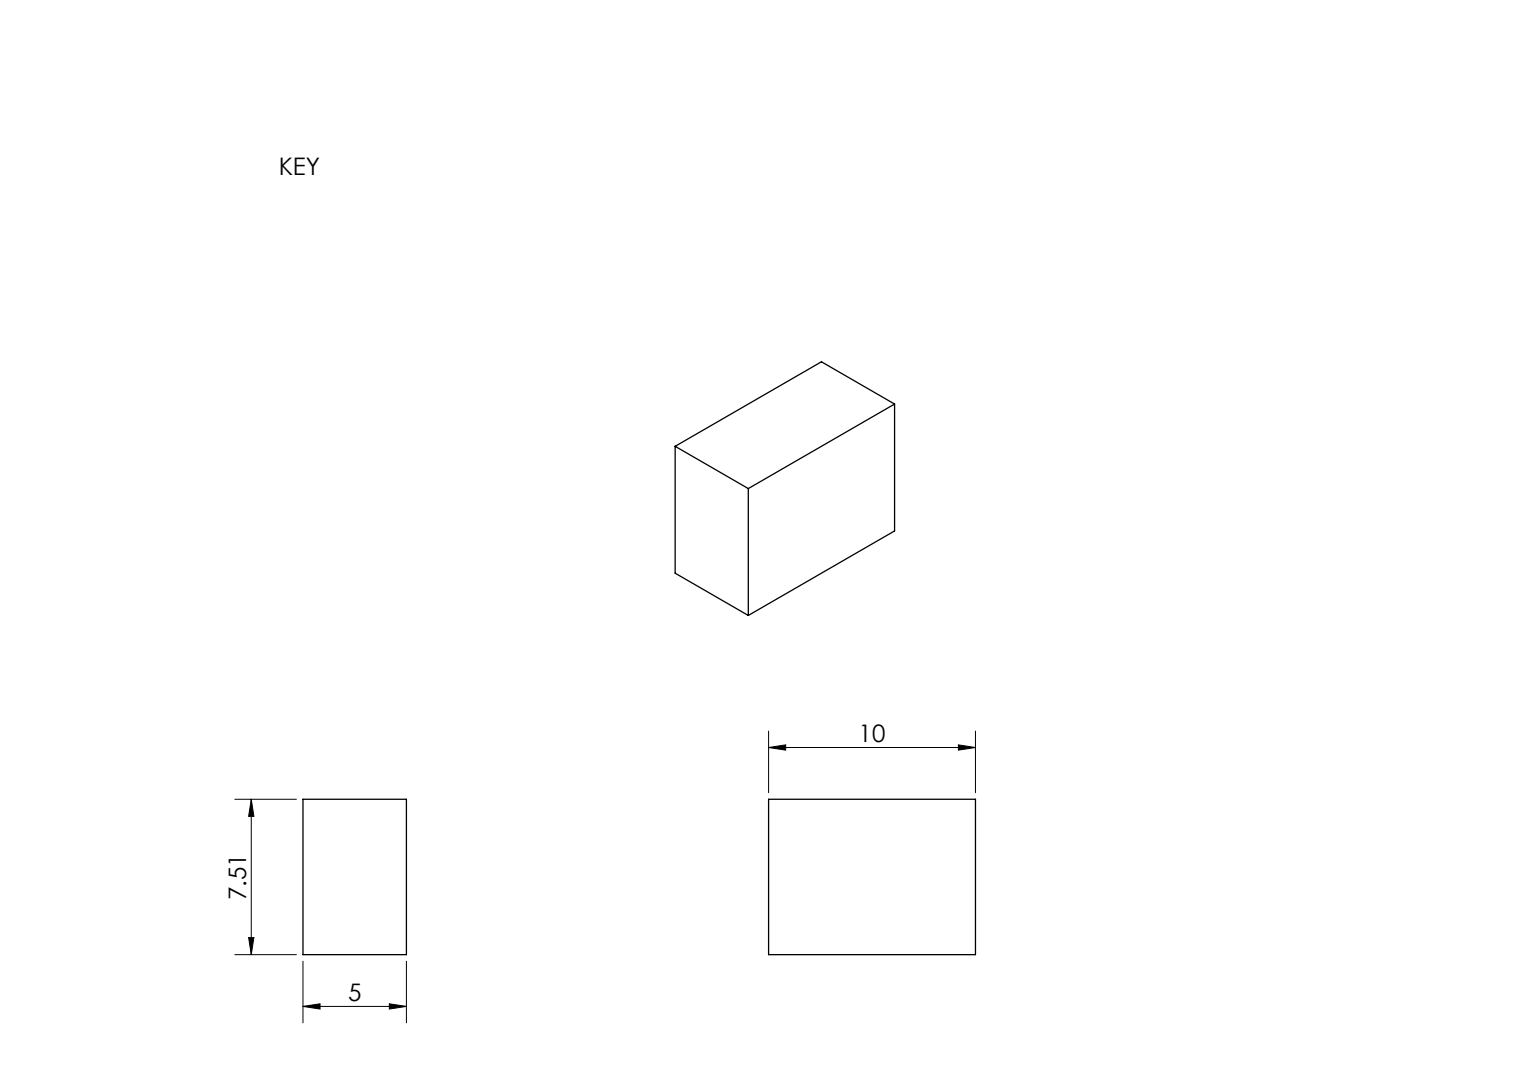
ISO-10303-21;
HEADER;
FILE_DESCRIPTION (('STEP AP214'),
    '1' );
FILE_NAME ('key.step',
    '2026-09-30T12:41:04',
    ( '' ),
    ( '' ),
    'SwSTEP 2.0',
    'SolidWorks 2026',
    '' );
FILE_SCHEMA (( 'AUTOMOTIVE_DESIGN' ));
ENDSEC;

DATA;
#157=PLANE ( 'NONE',  #35526 ) ;
#365=EDGE_LOOP ( 'NONE', ( #14092, #42320, #15486, #37127 ) ) ;
#413=DIRECTION ( 'NONE',  ( -5.778480238264233142E-17, 1.000000000000000000, 0.000000000000000000 ) ) ;
#1022=AXIS2_PLACEMENT_3D ( 'NONE', #2617, #17562, #47432 ) ;
#1267=CARTESIAN_POINT ( 'NONE',  ( -2.499999999999997780, 8.494897427831771708, -19.01812422950394676 ) ) ;
#1289=EDGE_CURVE ( 'NONE', #18460, #24623, #27553, .T. ) ;
#1398=SHAPE_REPRESENTATION_RELATIONSHIP ( 'NONE' , 'NONE' ,  #45973, #29206 ) ;
#2187=VECTOR ( 'NONE', #3487, 1000.000000000000000 ) ;
#2198=PRODUCT_DEFINITION_FORMATION_WITH_SPECIFIED_SOURCE ( 'ANY', '', #2652, .NOT_KNOWN. ) ;
#2310=CARTESIAN_POINT ( 'NONE',  ( -2.500000000000000000, 16.00000000000000000, 0.000000000000000000 ) ) ;
#2617=CARTESIAN_POINT ( 'NONE',  ( -1.066668064568189757E-15, -1.540743955509788682E-30, -10.00000000000000178 ) ) ;
#2652=PRODUCT ( 'key', 'key', '', ( #29200 ) ) ;
#3487=DIRECTION ( 'NONE',  ( 0.000000000000000000, 0.000000000000000000, 1.000000000000000000 ) ) ;
#3527=LINE ( 'NONE', #45605, #27393 ) ;
#3572=MANIFOLD_SOLID_BREP ( 'Boss-Extrude1', #23125 ) ;
#3667=DIRECTION ( 'NONE',  ( 1.000000000000000000, 0.000000000000000000, 0.000000000000000000 ) ) ;
#4293=ORIENTED_EDGE ( 'NONE', *, *, #28755, .F. ) ;
#5043=EDGE_CURVE ( 'NONE', #12792, #27374, #13841, .T. ) ;
#5142=EDGE_CURVE ( 'NONE', #35877, #12792, #6249, .T. ) ;
#5452=CARTESIAN_POINT ( 'NONE',  ( 2.500000000000000444, 8.494897427831771708, -10.00000000000000178 ) ) ;
#5458=CARTESIAN_POINT ( 'NONE',  ( -2.499999999999997780, 8.494897427831771708, 0.000000000000000000 ) ) ;
#5795=FILL_AREA_STYLE ('',( #43890 ) ) ;
#6249=LINE ( 'NONE', #17487, #28937 ) ;
#6466=ADVANCED_FACE ( 'NONE', ( #18755 ), #157, .T. ) ;
#6483=DIRECTION ( 'NONE',  ( 1.000000000000000000, 0.000000000000000000, 0.000000000000000000 ) ) ;
#6619=DIRECTION ( 'NONE',  ( 0.000000000000000000, 0.000000000000000000, 1.000000000000000000 ) ) ;
#6726=CARTESIAN_POINT ( 'NONE',  ( -2.500000000000000000, 16.00000000000000000, -10.00000000000000178 ) ) ;
#6853=CARTESIAN_POINT ( 'NONE',  ( 2.500000000000000000, 16.00000000000000000, -10.00000000000000178 ) ) ;
#7592=UNCERTAINTY_MEASURE_WITH_UNIT (LENGTH_MEASURE( 1.000000000000000082E-05 ), #10355, 'distance_accuracy_value', 'NONE');
#7732=VERTEX_POINT ( 'NONE', #2310 ) ;
#7917=DIRECTION ( 'NONE',  ( 0.000000000000000000, 0.000000000000000000, 1.000000000000000000 ) ) ;
#8710=FILL_AREA_STYLE_COLOUR ( '', #46663 ) ;
#8720=( NAMED_UNIT ( * ) PLANE_ANGLE_UNIT ( ) SI_UNIT ( $, .RADIAN. ) );
#8795=VECTOR ( 'NONE', #42481, 1000.000000000000000 ) ;
#8833=FACE_OUTER_BOUND ( 'NONE', #34894, .T. ) ;
#9469=EDGE_LOOP ( 'NONE', ( #26020, #32357, #4293, #17051 ) ) ;
#9475=CARTESIAN_POINT ( 'NONE',  ( -2.499999999999997780, 8.494897427831771708, -10.00000000000000178 ) ) ;
#9606=PLANE ( 'NONE',  #45530 ) ;
#9920=DIRECTION ( 'NONE',  ( 5.778480238264233142E-17, -1.000000000000000000, 0.000000000000000000 ) ) ;
#10097=PRODUCT_DEFINITION_SHAPE ( 'NONE', 'NONE',  #33713 ) ;
#10281=EDGE_CURVE ( 'NONE', #35877, #44453, #3527, .T. ) ;
#10355=( LENGTH_UNIT ( ) NAMED_UNIT ( * ) SI_UNIT ( .MILLI., .METRE. ) );
#10978=ORIENTED_EDGE ( 'NONE', *, *, #12662, .T. ) ;
#11636=AXIS2_PLACEMENT_3D ( 'NONE', #13959, #6619, #3667 ) ;
#12179=SURFACE_STYLE_FILL_AREA ( #31021 ) ;
#12616=ORIENTED_EDGE ( 'NONE', *, *, #32003, .T. ) ;
#12652=SURFACE_STYLE_USAGE ( .BOTH. , #17035 ) ;
#12662=EDGE_CURVE ( 'NONE', #7732, #44453, #22627, .T. ) ;
#12792=VERTEX_POINT ( 'NONE', #35333 ) ;
#12873=CARTESIAN_POINT ( 'NONE',  ( 2.500000000000000000, 16.00000000000000000, -19.01812422950394676 ) ) ;
#13045=MECHANICAL_DESIGN_GEOMETRIC_PRESENTATION_REPRESENTATION('',(#26317),#19277);
#13589=LINE ( 'NONE', #28528, #43402 ) ;
#13664=FACE_OUTER_BOUND ( 'NONE', #35395, .T. ) ;
#13841=LINE ( 'NONE', #6726, #26613 ) ;
#13959=CARTESIAN_POINT ( 'NONE',  ( 0.000000000000000000, 0.000000000000000000, 0.000000000000000000 ) ) ;
#14092=ORIENTED_EDGE ( 'NONE', *, *, #16713, .F. ) ;
#15105=CARTESIAN_POINT ( 'NONE',  ( 2.500000000000000000, 16.00000000000000000, -19.01812422950394676 ) ) ;
#15110=( NAMED_UNIT ( * ) SI_UNIT ( $, .STERADIAN. ) SOLID_ANGLE_UNIT ( ) );
#15121=( NAMED_UNIT ( * ) PLANE_ANGLE_UNIT ( ) SI_UNIT ( $, .RADIAN. ) );
#15222=ORIENTED_EDGE ( 'NONE', *, *, #21808, .F. ) ;
#15245=DIRECTION ( 'NONE',  ( 0.000000000000000000, -0.000000000000000000, 1.000000000000000000 ) ) ;
#15486=ORIENTED_EDGE ( 'NONE', *, *, #48449, .F. ) ;
#15867=ORIENTED_EDGE ( 'NONE', *, *, #48449, .T. ) ;
#16327=VECTOR ( 'NONE', #32096, 1000.000000000000000 ) ;
#16691=ORIENTED_EDGE ( 'NONE', *, *, #16713, .T. ) ;
#16713=EDGE_CURVE ( 'NONE', #18460, #35877, #28742, .T. ) ;
#17035=SURFACE_SIDE_STYLE ('',( #34917 ) ) ;
#17051=ORIENTED_EDGE ( 'NONE', *, *, #1289, .F. ) ;
#17147=CARTESIAN_POINT ( 'NONE',  ( -2.499999999999997780, 8.494897427831771708, 0.000000000000000000 ) ) ;
#17487=CARTESIAN_POINT ( 'NONE',  ( -2.500000000000000000, 16.00000000000000000, -10.00000000000000178 ) ) ;
#17562=DIRECTION ( 'NONE',  ( 0.000000000000000000, 0.000000000000000000, 1.000000000000000000 ) ) ;
#17803=CARTESIAN_POINT ( 'NONE',  ( 2.500000000000000000, 16.00000000000000000, 0.000000000000000000 ) ) ;
#18460=VERTEX_POINT ( 'NONE', #5452 ) ;
#18755=FACE_OUTER_BOUND ( 'NONE', #9469, .T. ) ;
#18951=ORIENTED_EDGE ( 'NONE', *, *, #5043, .F. ) ;
#19051=AXIS2_PLACEMENT_3D ( 'NONE', #23056, #41655, #15245 ) ;
#19277=( GEOMETRIC_REPRESENTATION_CONTEXT ( 3 ) GLOBAL_UNCERTAINTY_ASSIGNED_CONTEXT ( ( #41370 ) ) GLOBAL_UNIT_ASSIGNED_CONTEXT ( ( #26605, #38593, #15110 ) ) REPRESENTATION_CONTEXT ( 'NONE', 'WORKASPACE' ) );
#20227=PRESENTATION_STYLE_ASSIGNMENT (( #12652 ) ) ;
#21429=ADVANCED_FACE ( 'NONE', ( #39496 ), #9606, .T. ) ;
#21465=VECTOR ( 'NONE', #37561, 1000.000000000000000 ) ;
#21808=EDGE_CURVE ( 'NONE', #28899, #7732, #42566, .T. ) ;
#21979=ADVANCED_FACE ( 'NONE', ( #13664 ), #28597, .F. ) ;
#22627=LINE ( 'NONE', #38535, #21465 ) ;
#22933=( LENGTH_UNIT ( ) NAMED_UNIT ( * ) SI_UNIT ( .MILLI., .METRE. ) );
#23006=ADVANCED_FACE ( 'NONE', ( #8833 ), #37500, .T. ) ;
#23056=CARTESIAN_POINT ( 'NONE',  ( -2.500000000000000000, 16.00000000000000000, -19.01812422950394676 ) ) ;
#23125=CLOSED_SHELL ( 'NONE', ( #21429, #23006, #6466, #45957, #41020, #21979 ) ) ;
#23158=LINE ( 'NONE', #12873, #37778 ) ;
#23176=SURFACE_SIDE_STYLE ('',( #12179 ) ) ;
#23220=APPLICATION_CONTEXT ( 'automotive_design' ) ;
#23292=PLANE ( 'NONE',  #43452 ) ;
#24191=DIRECTION ( 'NONE',  ( -1.000000000000000000, -0.000000000000000000, -0.000000000000000000 ) ) ;
#24623=VERTEX_POINT ( 'NONE', #34440 ) ;
#24825=CARTESIAN_POINT ( 'NONE',  ( -2.499999999999997780, 8.494897427831771708, -10.00000000000000178 ) ) ;
#24871=MECHANICAL_DESIGN_GEOMETRIC_PRESENTATION_REPRESENTATION('',(#47547),#31952);
#25166=DIRECTION ( 'NONE',  ( -0.000000000000000000, 0.000000000000000000, 1.000000000000000000 ) ) ;
#26020=ORIENTED_EDGE ( 'NONE', *, *, #32003, .F. ) ;
#26317=STYLED_ITEM ( 'NONE', ( #27100 ), #3572 ) ;
#26605=( LENGTH_UNIT ( ) NAMED_UNIT ( * ) SI_UNIT ( .MILLI., .METRE. ) );
#26613=VECTOR ( 'NONE', #6483, 1000.000000000000000 ) ;
#26642=AXIS2_PLACEMENT_3D ( 'NONE', #35953, #25166, #32062 ) ;
#27100=PRESENTATION_STYLE_ASSIGNMENT (( #38109 ) ) ;
#27213=FACE_OUTER_BOUND ( 'NONE', #365, .T. ) ;
#27374=VERTEX_POINT ( 'NONE', #6853 ) ;
#27393=VECTOR ( 'NONE', #7917, 1000.000000000000000 ) ;
#27553=LINE ( 'NONE', #42235, #8795 ) ;
#27657=ORIENTED_EDGE ( 'NONE', *, *, #21808, .T. ) ;
#27839=( NAMED_UNIT ( * ) SI_UNIT ( $, .STERADIAN. ) SOLID_ANGLE_UNIT ( ) );
#28024=DIRECTION ( 'NONE',  ( -1.000000000000000000, 0.000000000000000000, 0.000000000000000000 ) ) ;
#28273=VECTOR ( 'NONE', #40563, 1000.000000000000000 ) ;
#28528=CARTESIAN_POINT ( 'NONE',  ( 2.500000000000000000, 16.00000000000000000, -10.00000000000000178 ) ) ;
#28550=ORIENTED_EDGE ( 'NONE', *, *, #28755, .T. ) ;
#28597=PLANE ( 'NONE',  #1022 ) ;
#28742=LINE ( 'NONE', #24825, #42627 ) ;
#28755=EDGE_CURVE ( 'NONE', #24623, #28899, #32728, .T. ) ;
#28899=VERTEX_POINT ( 'NONE', #41536 ) ;
#28937=VECTOR ( 'NONE', #32437, 1000.000000000000000 ) ;
#29200=PRODUCT_CONTEXT ( 'NONE', #39159, 'mechanical' ) ;
#29206=ADVANCED_BREP_SHAPE_REPRESENTATION ( '', ( #3572, #11636 ), #48316 ) ;
#29504=ORIENTED_EDGE ( 'NONE', *, *, #35411, .T. ) ;
#29819=ORIENTED_EDGE ( 'NONE', *, *, #5142, .T. ) ;
#30403=DIRECTION ( 'NONE',  ( 0.000000000000000000, -0.000000000000000000, -1.000000000000000000 ) ) ;
#31021=FILL_AREA_STYLE ('',( #8710 ) ) ;
#31076=CARTESIAN_POINT ( 'NONE',  ( -2.500000000000000000, 16.00000000000000000, 0.000000000000000000 ) ) ;
#31172=ORIENTED_EDGE ( 'NONE', *, *, #5142, .F. ) ;
#31434=CARTESIAN_POINT ( 'NONE',  ( -2.500000000000000000, 16.00000000000000000, -19.01812422950394676 ) ) ;
#31505=( NAMED_UNIT ( * ) SI_UNIT ( $, .STERADIAN. ) SOLID_ANGLE_UNIT ( ) );
#31755=ORIENTED_EDGE ( 'NONE', *, *, #5043, .T. ) ;
#31952=( GEOMETRIC_REPRESENTATION_CONTEXT ( 3 ) GLOBAL_UNCERTAINTY_ASSIGNED_CONTEXT ( ( #7592 ) ) GLOBAL_UNIT_ASSIGNED_CONTEXT ( ( #10355, #8720, #27839 ) ) REPRESENTATION_CONTEXT ( 'NONE', 'WORKASPACE' ) );
#32003=EDGE_CURVE ( 'NONE', #27374, #18460, #13589, .T. ) ;
#32062=DIRECTION ( 'NONE',  ( 1.000000000000000000, 0.000000000000000000, 0.000000000000000000 ) ) ;
#32096=DIRECTION ( 'NONE',  ( 1.000000000000000000, 0.000000000000000000, 0.000000000000000000 ) ) ;
#32357=ORIENTED_EDGE ( 'NONE', *, *, #42942, .T. ) ;
#32437=DIRECTION ( 'NONE',  ( -2.889240119132116694E-16, 1.000000000000000000, 0.000000000000000000 ) ) ;
#32728=LINE ( 'NONE', #17803, #28273 ) ;
#32754=FACE_OUTER_BOUND ( 'NONE', #42701, .T. ) ;
#32997=PLANE ( 'NONE',  #26642 ) ;
#33021=DIRECTION ( 'NONE',  ( 2.889240119132116694E-16, -1.000000000000000000, 0.000000000000000000 ) ) ;
#33041=PRODUCT_DEFINITION_CONTEXT ( 'detailed design', #23220, 'design' ) ;
#33221=DIRECTION ( 'NONE',  ( 1.000000000000000000, 5.778480238264233142E-17, -0.000000000000000000 ) ) ;
#33713=PRODUCT_DEFINITION ( 'UNKNOWN', '', #2198, #33041 ) ;
#34064=LINE ( 'NONE', #45096, #2187 ) ;
#34273=ORIENTED_EDGE ( 'NONE', *, *, #42942, .F. ) ;
#34440=CARTESIAN_POINT ( 'NONE',  ( 2.500000000000000444, 8.494897427831771708, 0.000000000000000000 ) ) ;
#34894=EDGE_LOOP ( 'NONE', ( #18951, #29504, #15222, #34273 ) ) ;
#34917=SURFACE_STYLE_FILL_AREA ( #5795 ) ;
#35333=CARTESIAN_POINT ( 'NONE',  ( -2.500000000000000000, 16.00000000000000000, -10.00000000000000178 ) ) ;
#35395=EDGE_LOOP ( 'NONE', ( #29819, #31755, #12616, #16691 ) ) ;
#35411=EDGE_CURVE ( 'NONE', #12792, #7732, #34064, .T. ) ;
#35526=AXIS2_PLACEMENT_3D ( 'NONE', #15105, #33221, #413 ) ;
#35877=VERTEX_POINT ( 'NONE', #9475 ) ;
#35953=CARTESIAN_POINT ( 'NONE',  ( 0.000000000000000000, 0.000000000000000000, 0.000000000000000000 ) ) ;
#37127=ORIENTED_EDGE ( 'NONE', *, *, #10281, .F. ) ;
#37353=EDGE_LOOP ( 'NONE', ( #31172, #39875, #45161, #43234 ) ) ;
#37386=COLOUR_RGB ( '', 0.40784314, 0.44705882, 0.49803922) ;
#37500=PLANE ( 'NONE',  #19051 ) ;
#37561=DIRECTION ( 'NONE',  ( 2.889240119132116694E-16, -1.000000000000000000, 0.000000000000000000 ) ) ;
#37778=VECTOR ( 'NONE', #42484, 1000.000000000000000 ) ;
#38109=SURFACE_STYLE_USAGE ( .BOTH. , #23176 ) ;
#38535=CARTESIAN_POINT ( 'NONE',  ( -2.500000000000000000, 16.00000000000000000, 0.000000000000000000 ) ) ;
#38593=( NAMED_UNIT ( * ) PLANE_ANGLE_UNIT ( ) SI_UNIT ( $, .RADIAN. ) );
#39159=APPLICATION_CONTEXT ( 'automotive_design' ) ;
#39242=DIRECTION ( 'NONE',  ( -1.000000000000000000, -2.889240119132116694E-16, 0.000000000000000000 ) ) ;
#39496=FACE_OUTER_BOUND ( 'NONE', #37353, .T. ) ;
#39875=ORIENTED_EDGE ( 'NONE', *, *, #10281, .T. ) ;
#40563=DIRECTION ( 'NONE',  ( -5.778480238264233142E-17, 1.000000000000000000, -0.000000000000000000 ) ) ;
#40897=VECTOR ( 'NONE', #24191, 1000.000000000000000 ) ;
#41020=ADVANCED_FACE ( 'NONE', ( #32754 ), #32997, .T. ) ;
#41370=UNCERTAINTY_MEASURE_WITH_UNIT (LENGTH_MEASURE( 1.000000000000000082E-05 ), #26605, 'distance_accuracy_value', 'NONE');
#41536=CARTESIAN_POINT ( 'NONE',  ( 2.500000000000000000, 16.00000000000000000, 0.000000000000000000 ) ) ;
#41655=DIRECTION ( 'NONE',  ( 0.000000000000000000, 1.000000000000000000, 0.000000000000000000 ) ) ;
#41859=UNCERTAINTY_MEASURE_WITH_UNIT (LENGTH_MEASURE( 1.000000000000000082E-05 ), #22933, 'distance_accuracy_value', 'NONE');
#41909=DIRECTION ( 'NONE',  ( 0.000000000000000000, -1.000000000000000000, 0.000000000000000000 ) ) ;
#42235=CARTESIAN_POINT ( 'NONE',  ( 2.500000000000000444, 8.494897427831771708, -19.01812422950394676 ) ) ;
#42320=ORIENTED_EDGE ( 'NONE', *, *, #1289, .T. ) ;
#42481=DIRECTION ( 'NONE',  ( 0.000000000000000000, 0.000000000000000000, 1.000000000000000000 ) ) ;
#42484=DIRECTION ( 'NONE',  ( 0.000000000000000000, 0.000000000000000000, 1.000000000000000000 ) ) ;
#42566=LINE ( 'NONE', #31076, #40897 ) ;
#42627=VECTOR ( 'NONE', #28024, 1000.000000000000000 ) ;
#42701=EDGE_LOOP ( 'NONE', ( #10978, #15867, #28550, #27657 ) ) ;
#42942=EDGE_CURVE ( 'NONE', #27374, #28899, #23158, .T. ) ;
#43234=ORIENTED_EDGE ( 'NONE', *, *, #35411, .F. ) ;
#43402=VECTOR ( 'NONE', #9920, 1000.000000000000000 ) ;
#43452=AXIS2_PLACEMENT_3D ( 'NONE', #1267, #41909, #30403 ) ;
#43585=LINE ( 'NONE', #17147, #16327 ) ;
#43890=FILL_AREA_STYLE_COLOUR ( '', #37386 ) ;
#44453=VERTEX_POINT ( 'NONE', #5458 ) ;
#44615=SHAPE_DEFINITION_REPRESENTATION ( #10097, #45973 ) ;
#45096=CARTESIAN_POINT ( 'NONE',  ( -2.500000000000000000, 16.00000000000000000, -19.01812422950394676 ) ) ;
#45161=ORIENTED_EDGE ( 'NONE', *, *, #12662, .F. ) ;
#45530=AXIS2_PLACEMENT_3D ( 'NONE', #31434, #39242, #33021 ) ;
#45605=CARTESIAN_POINT ( 'NONE',  ( -2.499999999999997780, 8.494897427831771708, -19.01812422950394676 ) ) ;
#45957=ADVANCED_FACE ( 'NONE', ( #27213 ), #23292, .T. ) ;
#45973=SHAPE_REPRESENTATION ( 'key', ( #11636 ), #48316 ) ;
#46663=COLOUR_RGB ( '', 0.40784314, 0.44705882, 0.49803922) ;
#47432=DIRECTION ( 'NONE',  ( 1.000000000000000000, 0.000000000000000000, 0.000000000000000000 ) ) ;
#47547=STYLED_ITEM ( 'NONE', ( #20227 ), #29206 ) ;
#48316=( GEOMETRIC_REPRESENTATION_CONTEXT ( 3 ) GLOBAL_UNCERTAINTY_ASSIGNED_CONTEXT ( ( #41859 ) ) GLOBAL_UNIT_ASSIGNED_CONTEXT ( ( #22933, #15121, #31505 ) ) REPRESENTATION_CONTEXT ( 'NONE', 'WORKASPACE' ) );
#48449=EDGE_CURVE ( 'NONE', #44453, #24623, #43585, .T. ) ;
ENDSEC;
END-ISO-10303-21;
